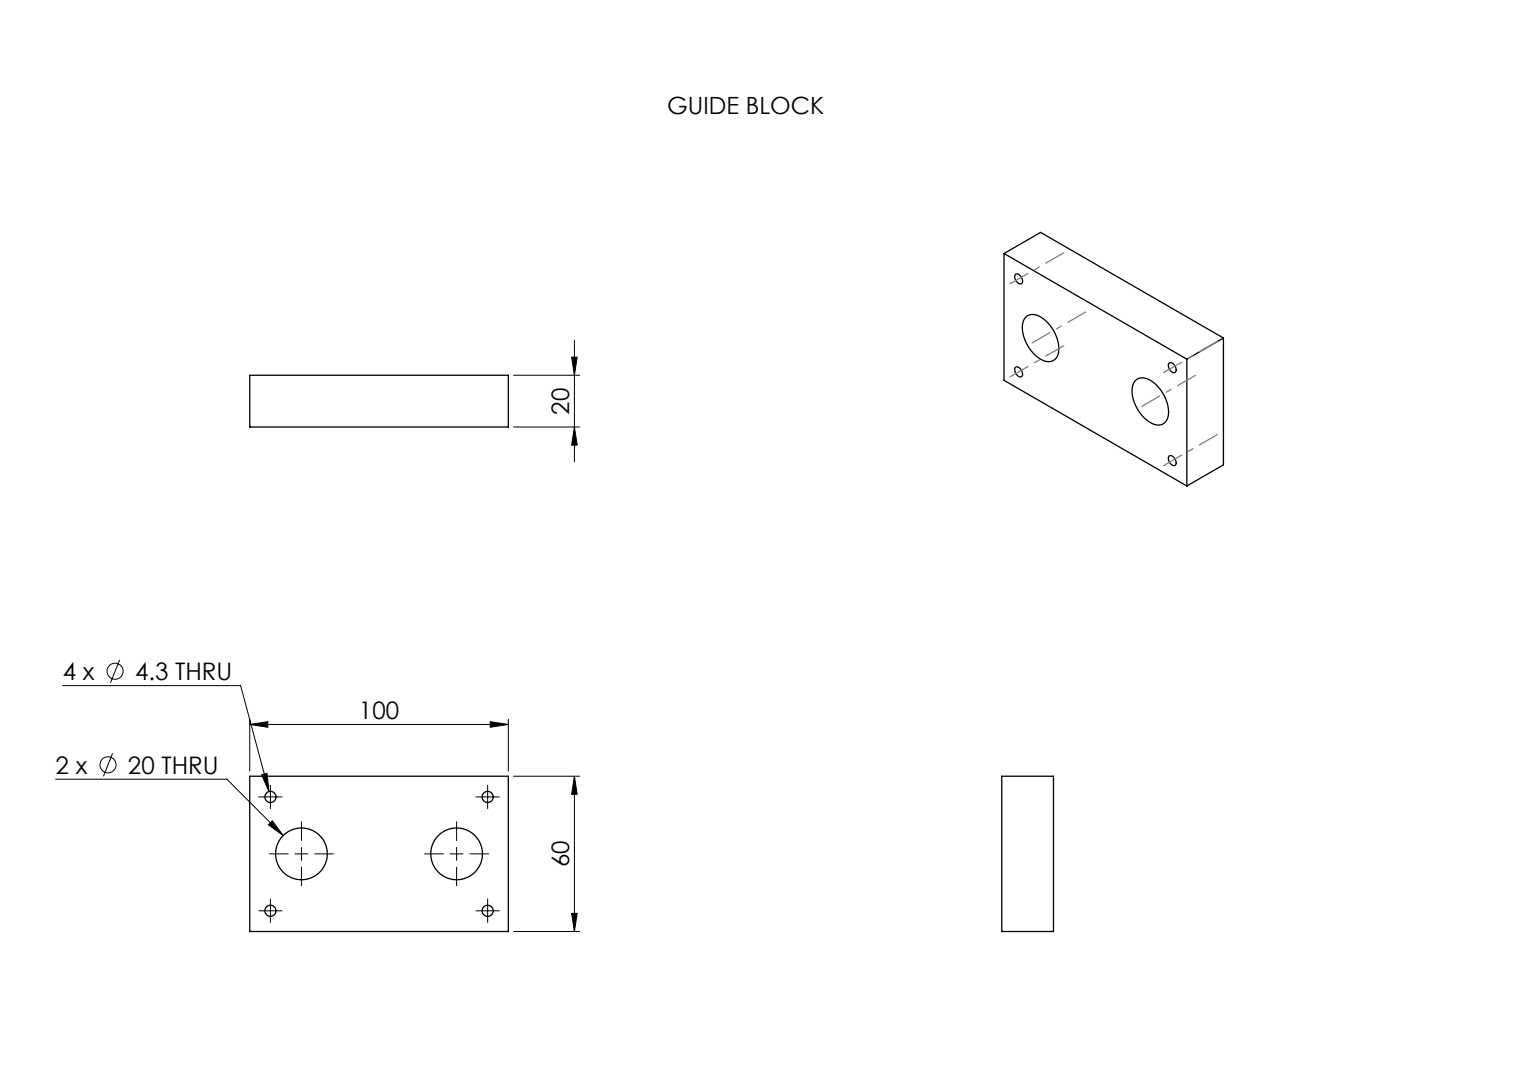
ISO-10303-21;
HEADER;
FILE_DESCRIPTION (('STEP AP214'),
    '1' );
FILE_NAME ('guide block.step',
    '2026-09-29T11:11:29',
    ( '' ),
    ( '' ),
    'SwSTEP 2.0',
    'SolidWorks 2026',
    '' );
FILE_SCHEMA (( 'AUTOMOTIVE_DESIGN' ));
ENDSEC;

DATA;
#8=ADVANCED_FACE ( 'NONE', ( #3264 ), #5944, .F. ) ;
#9=FACE_BOUND ( 'NONE', #6715, .T. ) ;
#15=ORIENTED_EDGE ( 'NONE', *, *, #7694, .T. ) ;
#24=ADVANCED_BREP_SHAPE_REPRESENTATION ( '', ( #85, #2554 ), #7190 ) ;
#41=EDGE_CURVE ( 'NONE', #505, #4648, #4851, .T. ) ;
#48=EDGE_LOOP ( 'NONE', ( #5523, #4308 ) ) ;
#49=CARTESIAN_POINT ( 'NONE',  ( -41.99999999999996447, -22.00000000000000000, 80.00000000000002842 ) ) ;
#67=CARTESIAN_POINT ( 'NONE',  ( 42.00000000000000711, -21.99999999999992184, 80.00000000000002842 ) ) ;
#74=AXIS2_PLACEMENT_3D ( 'NONE', #4907, #6141, #4116 ) ;
#80=DIRECTION ( 'NONE',  ( 1.000000000000000000, 0.000000000000000000, 0.000000000000000000 ) ) ;
#83=AXIS2_PLACEMENT_3D ( 'NONE', #2600, #8057, #1442 ) ;
#85=MANIFOLD_SOLID_BREP ( '\X2\00d8\X0\20.0 (20) Diameter Hole1', #4490 ) ;
#108=ORIENTED_EDGE ( 'NONE', *, *, #689, .F. ) ;
#120=VERTEX_POINT ( 'NONE', #6909 ) ;
#143=CIRCLE ( 'NONE', #4647, 9.999999999999998224 ) ;
#177=ADVANCED_FACE ( 'NONE', ( #4445 ), #1804, .F. ) ;
#184=LINE ( 'NONE', #7585, #2081 ) ;
#191=DIRECTION ( 'NONE',  ( -0.000000000000000000, 0.000000000000000000, 1.000000000000000000 ) ) ;
#212=SURFACE_SIDE_STYLE ('',( #6821 ) ) ;
#226=DIRECTION ( 'NONE',  ( -0.000000000000000000, -0.000000000000000000, -1.000000000000000000 ) ) ;
#231=CARTESIAN_POINT ( 'NONE',  ( -30.00000000000000000, 0.000000000000000000, 80.00000000000002842 ) ) ;
#234=EDGE_LOOP ( 'NONE', ( #2783, #7992, #7432, #4971 ) ) ;
#240=AXIS2_PLACEMENT_3D ( 'NONE', #1947, #6742, #7321 ) ;
#242=( GEOMETRIC_REPRESENTATION_CONTEXT ( 3 ) GLOBAL_UNCERTAINTY_ASSIGNED_CONTEXT ( ( #3453 ) ) GLOBAL_UNIT_ASSIGNED_CONTEXT ( ( #4314, #5632, #8331 ) ) REPRESENTATION_CONTEXT ( 'NONE', 'WORKASPACE' ) );
#250=EDGE_CURVE ( 'NONE', #6544, #5958, #4898, .T. ) ;
#273=DIRECTION ( 'NONE',  ( -0.000000000000000000, -0.000000000000000000, 1.000000000000000000 ) ) ;
#275=EDGE_CURVE ( 'NONE', #5958, #6544, #655, .T. ) ;
#293=EDGE_LOOP ( 'NONE', ( #5848, #7323 ) ) ;
#312=AXIS2_PLACEMENT_3D ( 'NONE', #7185, #3059, #1145 ) ;
#316=CARTESIAN_POINT ( 'NONE',  ( -39.84999999999998010, -22.00000000000000000, 80.00000000000002842 ) ) ;
#317=CARTESIAN_POINT ( 'NONE',  ( 39.85000000000002274, 21.99999999999992184, 60.00000000000002842 ) ) ;
#350=LINE ( 'NONE', #3185, #3142 ) ;
#368=AXIS2_PLACEMENT_3D ( 'NONE', #2667, #5963, #5335 ) ;
#380=LINE ( 'NONE', #8542, #1299 ) ;
#382=DIRECTION ( 'NONE',  ( -0.000000000000000000, 0.000000000000000000, 1.000000000000000000 ) ) ;
#406=DIRECTION ( 'NONE',  ( 1.000000000000000000, 0.000000000000000000, 0.000000000000000000 ) ) ;
#436=ORIENTED_EDGE ( 'NONE', *, *, #4043, .T. ) ;
#446=DIRECTION ( 'NONE',  ( 1.000000000000000000, 0.000000000000000000, 0.000000000000000000 ) ) ;
#459=DIRECTION ( 'NONE',  ( -0.000000000000000000, -0.000000000000000000, 1.000000000000000000 ) ) ;
#483=PLANE ( 'NONE',  #6432 ) ;
#490=( LENGTH_UNIT ( ) NAMED_UNIT ( * ) SI_UNIT ( .MILLI., .METRE. ) );
#504=EDGE_CURVE ( 'NONE', #3192, #4124, #958, .T. ) ;
#505=VERTEX_POINT ( 'NONE', #7187 ) ;
#517=AXIS2_PLACEMENT_3D ( 'NONE', #552, #1736, #7060 ) ;
#542=ORIENTED_EDGE ( 'NONE', *, *, #7814, .F. ) ;
#544=CARTESIAN_POINT ( 'NONE',  ( -39.99999999999999289, 1.224646799147353059E-15, 60.00000000000002842 ) ) ;
#545=CARTESIAN_POINT ( 'NONE',  ( -44.14999999999995595, 22.00000000000000000, 60.00000000000002842 ) ) ;
#549=CARTESIAN_POINT ( 'NONE',  ( -50.00000000000002842, -30.00000000000000000, 60.00000000000002842 ) ) ;
#552=CARTESIAN_POINT ( 'NONE',  ( 42.00000000000000711, 21.99999999999992184, 60.00000000000002842 ) ) ;
#560=AXIS2_PLACEMENT_3D ( 'NONE', #4014, #4102, #4307 ) ;
#576=CARTESIAN_POINT ( 'NONE',  ( 42.00000000000000711, -21.99999999999992184, 80.00000000000002842 ) ) ;
#608=UNCERTAINTY_MEASURE_WITH_UNIT (LENGTH_MEASURE( 1.000000000000000082E-05 ), #1837, 'distance_accuracy_value', 'NONE');
#623=DIRECTION ( 'NONE',  ( -1.000000000000000000, -0.000000000000000000, -0.000000000000000000 ) ) ;
#642=ORIENTED_EDGE ( 'NONE', *, *, #4452, .F. ) ;
#655=CIRCLE ( 'NONE', #1387, 2.149999999999985256 ) ;
#662=DIRECTION ( 'NONE',  ( 1.000000000000000000, 0.000000000000000000, 0.000000000000000000 ) ) ;
#667=FACE_BOUND ( 'NONE', #7929, .T. ) ;
#670=DIRECTION ( 'NONE',  ( -0.000000000000000000, -0.000000000000000000, 1.000000000000000000 ) ) ;
#680=ORIENTED_EDGE ( 'NONE', *, *, #275, .T. ) ;
#684=CARTESIAN_POINT ( 'NONE',  ( 29.99999999999997158, 1.102182119232617753E-14, 80.00000000000002842 ) ) ;
#689=EDGE_CURVE ( 'NONE', #4311, #8113, #1014, .T. ) ;
#703=LINE ( 'NONE', #3322, #4754 ) ;
#738=ORIENTED_EDGE ( 'NONE', *, *, #5306, .T. ) ;
#770=ORIENTED_EDGE ( 'NONE', *, *, #6382, .T. ) ;
#779=EDGE_LOOP ( 'NONE', ( #8638, #5179, #3636, #2635 ) ) ;
#831=DIRECTION ( 'NONE',  ( -0.000000000000000000, 0.000000000000000000, 1.000000000000000000 ) ) ;
#851=ORIENTED_EDGE ( 'NONE', *, *, #4407, .F. ) ;
#865=( GEOMETRIC_REPRESENTATION_CONTEXT ( 3 ) GLOBAL_UNCERTAINTY_ASSIGNED_CONTEXT ( ( #8028 ) ) GLOBAL_UNIT_ASSIGNED_CONTEXT ( ( #490, #6581, #1919 ) ) REPRESENTATION_CONTEXT ( 'NONE', 'WORKASPACE' ) );
#871=CARTESIAN_POINT ( 'NONE',  ( 50.00000000000002842, 30.00000000000000000, 80.00000000000002842 ) ) ;
#874=CARTESIAN_POINT ( 'NONE',  ( -41.99999999999996447, 22.00000000000000000, 60.00000000000002842 ) ) ;
#878=CIRCLE ( 'NONE', #6363, 2.149999999999985256 ) ;
#890=LINE ( 'NONE', #8264, #2347 ) ;
#894=CARTESIAN_POINT ( 'NONE',  ( 19.99999999999997513, 1.224646799147352901E-14, 60.00000000000002842 ) ) ;
#904=ADVANCED_FACE ( 'NONE', ( #6066 ), #8012, .F. ) ;
#923=VERTEX_POINT ( 'NONE', #545 ) ;
#936=FACE_OUTER_BOUND ( 'NONE', #5015, .T. ) ;
#938=DIRECTION ( 'NONE',  ( -0.000000000000000000, -0.000000000000000000, -1.000000000000000000 ) ) ;
#949=DIRECTION ( 'NONE',  ( -0.000000000000000000, -0.000000000000000000, 1.000000000000000000 ) ) ;
#958=CIRCLE ( 'NONE', #517, 2.149999999999985256 ) ;
#994=ORIENTED_EDGE ( 'NONE', *, *, #4575, .T. ) ;
#1001=DIRECTION ( 'NONE',  ( 1.000000000000000000, 0.000000000000000000, 0.000000000000000000 ) ) ;
#1014=CIRCLE ( 'NONE', #1437, 9.999999999999994671 ) ;
#1030=AXIS2_PLACEMENT_3D ( 'NONE', #3905, #1084, #4520 ) ;
#1060=VECTOR ( 'NONE', #1897, 1000.000000000000000 ) ;
#1084=DIRECTION ( 'NONE',  ( -0.000000000000000000, 0.000000000000000000, 1.000000000000000000 ) ) ;
#1087=VECTOR ( 'NONE', #7029, 1000.000000000000000 ) ;
#1104=DIRECTION ( 'NONE',  ( 1.000000000000000000, 0.000000000000000000, 0.000000000000000000 ) ) ;
#1108=LINE ( 'NONE', #2483, #4639 ) ;
#1109=LINE ( 'NONE', #3152, #4900 ) ;
#1130=CIRCLE ( 'NONE', #6474, 2.149999999999985256 ) ;
#1131=DIRECTION ( 'NONE',  ( -0.000000000000000000, 0.000000000000000000, 1.000000000000000000 ) ) ;
#1136=ORIENTED_EDGE ( 'NONE', *, *, #41, .T. ) ;
#1145=DIRECTION ( 'NONE',  ( 1.000000000000000000, 0.000000000000000000, 0.000000000000000000 ) ) ;
#1159=LINE ( 'NONE', #7780, #1087 ) ;
#1168=CARTESIAN_POINT ( 'NONE',  ( 44.14999999999999147, 21.99999999999992184, 60.00000000000002842 ) ) ;
#1200=PLANE ( 'NONE',  #368 ) ;
#1205=LINE ( 'NONE', #5255, #2854 ) ;
#1230=DIRECTION ( 'NONE',  ( 0.000000000000000000, -1.000000000000000000, 0.000000000000000000 ) ) ;
#1248=SHAPE_REPRESENTATION_RELATIONSHIP ( 'NONE' , 'NONE' ,  #4396, #24 ) ;
#1276=MECHANICAL_DESIGN_GEOMETRIC_PRESENTATION_REPRESENTATION('',(#2556),#865);
#1291=DIRECTION ( 'NONE',  ( 0.000000000000000000, -1.000000000000000000, 0.000000000000000000 ) ) ;
#1297=VERTEX_POINT ( 'NONE', #2924 ) ;
#1299=VECTOR ( 'NONE', #459, 1000.000000000000000 ) ;
#1350=ORIENTED_EDGE ( 'NONE', *, *, #250, .T. ) ;
#1371=ORIENTED_EDGE ( 'NONE', *, *, #3878, .F. ) ;
#1375=CYLINDRICAL_SURFACE ( 'NONE', #4181, 9.999999999999994671 ) ;
#1376=CARTESIAN_POINT ( 'NONE',  ( -40.00000000000000000, 1.224646799147353454E-15, 80.00000000000002842 ) ) ;
#1381=FILL_AREA_STYLE_COLOUR ( '', #8474 ) ;
#1383=CARTESIAN_POINT ( 'NONE',  ( -41.99999999999996447, 22.00000000000000000, 80.00000000000002842 ) ) ;
#1387=AXIS2_PLACEMENT_3D ( 'NONE', #3825, #5720, #7090 ) ;
#1416=FACE_BOUND ( 'NONE', #1448, .T. ) ;
#1418=EDGE_CURVE ( 'NONE', #7457, #2517, #6025, .T. ) ;
#1421=EDGE_CURVE ( 'NONE', #2540, #2072, #5423, .T. ) ;
#1428=PLANE ( 'NONE',  #6426 ) ;
#1434=VERTEX_POINT ( 'NONE', #549 ) ;
#1437=AXIS2_PLACEMENT_3D ( 'NONE', #3049, #3701, #6381 ) ;
#1442=DIRECTION ( 'NONE',  ( 0.000000000000000000, -0.000000000000000000, 1.000000000000000000 ) ) ;
#1444=ADVANCED_FACE ( 'NONE', ( #7394 ), #5354, .F. ) ;
#1448=EDGE_LOOP ( 'NONE', ( #7819, #5270 ) ) ;
#1506=AXIS2_PLACEMENT_3D ( 'NONE', #1715, #5676, #1001 ) ;
#1550=DIRECTION ( 'NONE',  ( -0.000000000000000000, -0.000000000000000000, 1.000000000000000000 ) ) ;
#1576=PRODUCT_DEFINITION ( 'UNKNOWN', '', #3409, #8552 ) ;
#1595=CYLINDRICAL_SURFACE ( 'NONE', #74, 9.999999999999994671 ) ;
#1627=ORIENTED_EDGE ( 'NONE', *, *, #6127, .F. ) ;
#1635=VECTOR ( 'NONE', #5981, 1000.000000000000000 ) ;
#1685=CARTESIAN_POINT ( 'NONE',  ( -50.00000000000002842, -30.00000000000000000, 60.00000000000002842 ) ) ;
#1707=DIRECTION ( 'NONE',  ( 0.000000000000000000, 0.000000000000000000, 1.000000000000000000 ) ) ;
#1712=AXIS2_PLACEMENT_3D ( 'NONE', #6266, #5601, #7672 ) ;
#1715=CARTESIAN_POINT ( 'NONE',  ( -41.99999999999996447, 22.00000000000000000, 80.00000000000002842 ) ) ;
#1736=DIRECTION ( 'NONE',  ( -0.000000000000000000, 0.000000000000000000, 1.000000000000000000 ) ) ;
#1737=DIRECTION ( 'NONE',  ( 1.000000000000000000, 0.000000000000000000, 0.000000000000000000 ) ) ;
#1745=ORIENTED_EDGE ( 'NONE', *, *, #41, .F. ) ;
#1761=ORIENTED_EDGE ( 'NONE', *, *, #5886, .T. ) ;
#1778=LINE ( 'NONE', #4007, #5943 ) ;
#1780=CARTESIAN_POINT ( 'NONE',  ( 42.00000000000000711, -21.99999999999992184, 80.00000000000002842 ) ) ;
#1802=MECHANICAL_DESIGN_GEOMETRIC_PRESENTATION_REPRESENTATION('',(#7848),#242);
#1804=CYLINDRICAL_SURFACE ( 'NONE', #1506, 2.149999999999985256 ) ;
#1811=ORIENTED_EDGE ( 'NONE', *, *, #5412, .T. ) ;
#1818=ADVANCED_FACE ( 'NONE', ( #6047 ), #1375, .F. ) ;
#1836=ADVANCED_FACE ( 'NONE', ( #7327, #2622, #667, #5251, #9, #3418, #8694 ), #1200, .T. ) ;
#1837=( LENGTH_UNIT ( ) NAMED_UNIT ( * ) SI_UNIT ( .MILLI., .METRE. ) );
#1854=EDGE_CURVE ( 'NONE', #7457, #1434, #7240, .T. ) ;
#1886=ORIENTED_EDGE ( 'NONE', *, *, #4542, .F. ) ;
#1887=VERTEX_POINT ( 'NONE', #1954 ) ;
#1894=ORIENTED_EDGE ( 'NONE', *, *, #4940, .T. ) ;
#1897=DIRECTION ( 'NONE',  ( 1.000000000000000000, 0.000000000000000000, 0.000000000000000000 ) ) ;
#1911=AXIS2_PLACEMENT_3D ( 'NONE', #3063, #5945, #1737 ) ;
#1919=( NAMED_UNIT ( * ) SI_UNIT ( $, .STERADIAN. ) SOLID_ANGLE_UNIT ( ) );
#1929=DIRECTION ( 'NONE',  ( -0.000000000000000000, -0.000000000000000000, 1.000000000000000000 ) ) ;
#1947=CARTESIAN_POINT ( 'NONE',  ( 29.99999999999997158, 1.102182119232617753E-14, 60.00000000000002842 ) ) ;
#1950=ORIENTED_EDGE ( 'NONE', *, *, #3451, .T. ) ;
#1954=CARTESIAN_POINT ( 'NONE',  ( 44.14999999999999147, 21.99999999999992184, 80.00000000000002842 ) ) ;
#1988=EDGE_CURVE ( 'NONE', #4697, #4311, #890, .T. ) ;
#2007=ORIENTED_EDGE ( 'NONE', *, *, #3451, .F. ) ;
#2008=DIRECTION ( 'NONE',  ( -0.000000000000000000, -0.000000000000000000, 1.000000000000000000 ) ) ;
#2014=EDGE_LOOP ( 'NONE', ( #6914, #542 ) ) ;
#2020=DIRECTION ( 'NONE',  ( 1.000000000000000000, 0.000000000000000000, 0.000000000000000000 ) ) ;
#2021=DIRECTION ( 'NONE',  ( -0.000000000000000000, 0.000000000000000000, 1.000000000000000000 ) ) ;
#2026=ADVANCED_FACE ( 'NONE', ( #6094 ), #1595, .F. ) ;
#2037=CARTESIAN_POINT ( 'NONE',  ( 39.85000000000002274, 21.99999999999992184, 80.00000000000002842 ) ) ;
#2051=SURFACE_STYLE_FILL_AREA ( #5299 ) ;
#2071=ORIENTED_EDGE ( 'NONE', *, *, #4679, .T. ) ;
#2072=VERTEX_POINT ( 'NONE', #5467 ) ;
#2081=VECTOR ( 'NONE', #226, 1000.000000000000000 ) ;
#2088=ORIENTED_EDGE ( 'NONE', *, *, #4214, .T. ) ;
#2108=ORIENTED_EDGE ( 'NONE', *, *, #5306, .F. ) ;
#2120=FILL_AREA_STYLE_COLOUR ( '', #3766 ) ;
#2129=CIRCLE ( 'NONE', #2684, 2.149999999999985256 ) ;
#2187=ORIENTED_EDGE ( 'NONE', *, *, #4214, .F. ) ;
#2189=ORIENTED_EDGE ( 'NONE', *, *, #504, .F. ) ;
#2229=CARTESIAN_POINT ( 'NONE',  ( 42.00000000000000711, 21.99999999999992184, 80.00000000000002842 ) ) ;
#2252=DIRECTION ( 'NONE',  ( -0.000000000000000000, -0.000000000000000000, -1.000000000000000000 ) ) ;
#2277=LINE ( 'NONE', #3144, #7975 ) ;
#2286=EDGE_CURVE ( 'NONE', #5578, #7382, #6687, .T. ) ;
#2302=VERTEX_POINT ( 'NONE', #316 ) ;
#2304=CIRCLE ( 'NONE', #5111, 9.999999999999994671 ) ;
#2313=EDGE_CURVE ( 'NONE', #1434, #120, #8639, .T. ) ;
#2323=VERTEX_POINT ( 'NONE', #2400 ) ;
#2347=VECTOR ( 'NONE', #1550, 1000.000000000000000 ) ;
#2386=DIRECTION ( 'NONE',  ( 1.000000000000000000, 0.000000000000000000, 0.000000000000000000 ) ) ;
#2400=CARTESIAN_POINT ( 'NONE',  ( 39.85000000000002274, -21.99999999999992184, 80.00000000000002842 ) ) ;
#2404=CARTESIAN_POINT ( 'NONE',  ( -39.84999999999998010, 22.00000000000000000, 60.00000000000002842 ) ) ;
#2413=DIRECTION ( 'NONE',  ( 1.000000000000000000, 0.000000000000000000, 0.000000000000000000 ) ) ;
#2437=CARTESIAN_POINT ( 'NONE',  ( -30.00000000000000000, 0.000000000000000000, 60.00000000000002842 ) ) ;
#2442=CARTESIAN_POINT ( 'NONE',  ( 44.14999999999999147, -21.99999999999992184, 80.00000000000002842 ) ) ;
#2446=CIRCLE ( 'NONE', #1030, 9.999999999999994671 ) ;
#2447=ORIENTED_EDGE ( 'NONE', *, *, #4575, .F. ) ;
#2476=VECTOR ( 'NONE', #6589, 1000.000000000000000 ) ;
#2480=CYLINDRICAL_SURFACE ( 'NONE', #312, 2.149999999999985256 ) ;
#2483=CARTESIAN_POINT ( 'NONE',  ( 44.14999999999999147, 21.99999999999992184, 80.00000000000002842 ) ) ;
#2490=EDGE_CURVE ( 'NONE', #2072, #2323, #4529, .T. ) ;
#2496=EDGE_CURVE ( 'NONE', #923, #7483, #380, .T. ) ;
#2506=VERTEX_POINT ( 'NONE', #544 ) ;
#2517=VERTEX_POINT ( 'NONE', #8582 ) ;
#2540=VERTEX_POINT ( 'NONE', #4403 ) ;
#2545=EDGE_LOOP ( 'NONE', ( #6333, #1745, #2108, #1761 ) ) ;
#2554=AXIS2_PLACEMENT_3D ( 'NONE', #7787, #1707, #3692 ) ;
#2556=STYLED_ITEM ( 'NONE', ( #4564 ), #24 ) ;
#2593=ORIENTED_EDGE ( 'NONE', *, *, #8199, .F. ) ;
#2597=DIRECTION ( 'NONE',  ( -0.000000000000000000, -0.000000000000000000, 1.000000000000000000 ) ) ;
#2600=CARTESIAN_POINT ( 'NONE',  ( -50.00000000000002842, -30.00000000000000000, 80.00000000000002842 ) ) ;
#2604=ORIENTED_EDGE ( 'NONE', *, *, #275, .F. ) ;
#2618=FACE_BOUND ( 'NONE', #8172, .T. ) ;
#2622=FACE_BOUND ( 'NONE', #7527, .T. ) ;
#2628=( NAMED_UNIT ( * ) SI_UNIT ( $, .STERADIAN. ) SOLID_ANGLE_UNIT ( ) );
#2635=ORIENTED_EDGE ( 'NONE', *, *, #7694, .F. ) ;
#2636=ORIENTED_EDGE ( 'NONE', *, *, #6281, .F. ) ;
#2667=CARTESIAN_POINT ( 'NONE',  ( 0.000000000000000000, 0.000000000000000000, 80.00000000000002842 ) ) ;
#2670=CARTESIAN_POINT ( 'NONE',  ( -39.84999999999998010, -22.00000000000000000, 80.00000000000002842 ) ) ;
#2680=EDGE_LOOP ( 'NONE', ( #738, #1950, #2716, #5385 ) ) ;
#2684=AXIS2_PLACEMENT_3D ( 'NONE', #7741, #7080, #446 ) ;
#2712=DIRECTION ( 'NONE',  ( -0.000000000000000000, -0.000000000000000000, 1.000000000000000000 ) ) ;
#2716=ORIENTED_EDGE ( 'NONE', *, *, #4452, .T. ) ;
#2745=ADVANCED_FACE ( 'NONE', ( #6021 ), #7434, .F. ) ;
#2753=DIRECTION ( 'NONE',  ( -0.000000000000000000, -0.000000000000000000, 1.000000000000000000 ) ) ;
#2783=ORIENTED_EDGE ( 'NONE', *, *, #4976, .F. ) ;
#2794=SHAPE_DEFINITION_REPRESENTATION ( #8394, #4396 ) ;
#2819=ORIENTED_EDGE ( 'NONE', *, *, #4417, .F. ) ;
#2824=AXIS2_PLACEMENT_3D ( 'NONE', #8000, #2712, #8617 ) ;
#2847=DIRECTION ( 'NONE',  ( -0.000000000000000000, -0.000000000000000000, 1.000000000000000000 ) ) ;
#2854=VECTOR ( 'NONE', #7379, 1000.000000000000000 ) ;
#2868=CIRCLE ( 'NONE', #4543, 2.149999999999985256 ) ;
#2896=ORIENTED_EDGE ( 'NONE', *, *, #5886, .F. ) ;
#2913=ORIENTED_EDGE ( 'NONE', *, *, #8104, .F. ) ;
#2924=CARTESIAN_POINT ( 'NONE',  ( -50.00000000000002842, 30.00000000000000000, 60.00000000000002842 ) ) ;
#2930=EDGE_CURVE ( 'NONE', #5183, #1887, #2868, .T. ) ;
#2934=CARTESIAN_POINT ( 'NONE',  ( -50.00000000000002842, 30.00000000000000000, 80.00000000000002842 ) ) ;
#2952=AXIS2_PLACEMENT_3D ( 'NONE', #3355, #5272, #6641 ) ;
#2957=PRESENTATION_STYLE_ASSIGNMENT (( #4802 ) ) ;
#3017=CARTESIAN_POINT ( 'NONE',  ( -39.84999999999998010, 22.00000000000000000, 80.00000000000002842 ) ) ;
#3049=CARTESIAN_POINT ( 'NONE',  ( 29.99999999999997158, 1.102182119232617753E-14, 80.00000000000002842 ) ) ;
#3054=ORIENTED_EDGE ( 'NONE', *, *, #8104, .T. ) ;
#3059=DIRECTION ( 'NONE',  ( -0.000000000000000000, -0.000000000000000000, 1.000000000000000000 ) ) ;
#3063=CARTESIAN_POINT ( 'NONE',  ( -30.00000000000000000, 0.000000000000000000, 80.00000000000002842 ) ) ;
#3064=DIRECTION ( 'NONE',  ( -0.000000000000000000, -0.000000000000000000, 1.000000000000000000 ) ) ;
#3116=DIRECTION ( 'NONE',  ( -1.000000000000000000, 0.000000000000000000, 0.000000000000000000 ) ) ;
#3138=EDGE_CURVE ( 'NONE', #2506, #6156, #2446, .T. ) ;
#3142=VECTOR ( 'NONE', #5736, 1000.000000000000000 ) ;
#3144=CARTESIAN_POINT ( 'NONE',  ( -50.00000000000002842, 30.00000000000000000, 80.00000000000002842 ) ) ;
#3147=AXIS2_PLACEMENT_3D ( 'NONE', #5871, #5914, #3976 ) ;
#3152=CARTESIAN_POINT ( 'NONE',  ( 50.00000000000002842, 30.00000000000000000, 60.00000000000002842 ) ) ;
#3185=CARTESIAN_POINT ( 'NONE',  ( 39.85000000000002274, 21.99999999999992184, 80.00000000000002842 ) ) ;
#3192=VERTEX_POINT ( 'NONE', #1168 ) ;
#3203=LINE ( 'NONE', #7912, #4711 ) ;
#3246=( NAMED_UNIT ( * ) PLANE_ANGLE_UNIT ( ) SI_UNIT ( $, .RADIAN. ) );
#3264=FACE_OUTER_BOUND ( 'NONE', #7296, .T. ) ;
#3291=DIRECTION ( 'NONE',  ( 1.000000000000000000, 0.000000000000000000, 0.000000000000000000 ) ) ;
#3295=SURFACE_SIDE_STYLE ('',( #2051 ) ) ;
#3308=AXIS2_PLACEMENT_3D ( 'NONE', #6496, #5711, #406 ) ;
#3322=CARTESIAN_POINT ( 'NONE',  ( 50.00000000000002842, 30.00000000000000000, 80.00000000000002842 ) ) ;
#3326=CYLINDRICAL_SURFACE ( 'NONE', #8419, 2.149999999999985256 ) ;
#3349=ADVANCED_FACE ( 'NONE', ( #5970 ), #1428, .F. ) ;
#3355=CARTESIAN_POINT ( 'NONE',  ( -30.00000000000000000, 0.000000000000000000, 80.00000000000002842 ) ) ;
#3380=CARTESIAN_POINT ( 'NONE',  ( -50.00000000000002842, 30.00000000000000000, 80.00000000000002842 ) ) ;
#3384=EDGE_CURVE ( 'NONE', #5890, #7483, #4317, .T. ) ;
#3385=ORIENTED_EDGE ( 'NONE', *, *, #5412, .F. ) ;
#3409=PRODUCT_DEFINITION_FORMATION_WITH_SPECIFIED_SOURCE ( 'ANY', '', #7676, .NOT_KNOWN. ) ;
#3418=FACE_BOUND ( 'NONE', #293, .T. ) ;
#3451=EDGE_CURVE ( 'NONE', #505, #4683, #2277, .T. ) ;
#3453=UNCERTAINTY_MEASURE_WITH_UNIT (LENGTH_MEASURE( 1.000000000000000082E-05 ), #4314, 'distance_accuracy_value', 'NONE');
#3494=CIRCLE ( 'NONE', #240, 9.999999999999994671 ) ;
#3509=CARTESIAN_POINT ( 'NONE',  ( 50.00000000000002842, 30.00000000000000000, 60.00000000000002842 ) ) ;
#3527=ORIENTED_EDGE ( 'NONE', *, *, #4675, .T. ) ;
#3536=AXIS2_PLACEMENT_3D ( 'NONE', #4910, #191, #6314 ) ;
#3546=CYLINDRICAL_SURFACE ( 'NONE', #4500, 2.149999999999985256 ) ;
#3548=DIRECTION ( 'NONE',  ( -0.000000000000000000, -0.000000000000000000, 1.000000000000000000 ) ) ;
#3561=CIRCLE ( 'NONE', #8484, 2.149999999999985256 ) ;
#3594=LINE ( 'NONE', #6098, #3719 ) ;
#3596=DIRECTION ( 'NONE',  ( -0.000000000000000000, -0.000000000000000000, 1.000000000000000000 ) ) ;
#3630=CARTESIAN_POINT ( 'NONE',  ( -39.99999999999999289, 1.224646799147352862E-15, 80.00000000000002842 ) ) ;
#3636=ORIENTED_EDGE ( 'NONE', *, *, #689, .T. ) ;
#3651=ADVANCED_FACE ( 'NONE', ( #7021 ), #4957, .F. ) ;
#3692=DIRECTION ( 'NONE',  ( 1.000000000000000000, 0.000000000000000000, 0.000000000000000000 ) ) ;
#3701=DIRECTION ( 'NONE',  ( -0.000000000000000000, -0.000000000000000000, 1.000000000000000000 ) ) ;
#3717=CYLINDRICAL_SURFACE ( 'NONE', #8169, 2.149999999999985256 ) ;
#3719=VECTOR ( 'NONE', #2847, 1000.000000000000000 ) ;
#3766=COLOUR_RGB ( '', 0.09019608, 0.27058824, 0.51372549) ;
#3798=VECTOR ( 'NONE', #273, 1000.000000000000000 ) ;
#3823=ORIENTED_EDGE ( 'NONE', *, *, #7586, .T. ) ;
#3825=CARTESIAN_POINT ( 'NONE',  ( -41.99999999999996447, -22.00000000000000000, 60.00000000000002842 ) ) ;
#3835=CARTESIAN_POINT ( 'NONE',  ( -44.14999999999995595, -22.00000000000000000, 80.00000000000002842 ) ) ;
#3836=ADVANCED_FACE ( 'NONE', ( #6798 ), #3546, .F. ) ;
#3838=CARTESIAN_POINT ( 'NONE',  ( -20.00000000000000355, 0.000000000000000000, 60.00000000000002842 ) ) ;
#3855=FACE_OUTER_BOUND ( 'NONE', #2545, .T. ) ;
#3875=DIRECTION ( 'NONE',  ( 1.000000000000000000, 0.000000000000000000, 0.000000000000000000 ) ) ;
#3878=EDGE_CURVE ( 'NONE', #6156, #7382, #7545, .T. ) ;
#3895=DIRECTION ( 'NONE',  ( -0.000000000000000000, -0.000000000000000000, -1.000000000000000000 ) ) ;
#3904=EDGE_LOOP ( 'NONE', ( #8667, #2896, #5028, #8192 ) ) ;
#3905=CARTESIAN_POINT ( 'NONE',  ( -30.00000000000000000, 0.000000000000000000, 60.00000000000002842 ) ) ;
#3932=CARTESIAN_POINT ( 'NONE',  ( -41.99999999999996447, -22.00000000000000000, 80.00000000000002842 ) ) ;
#3938=CIRCLE ( 'NONE', #2824, 2.149999999999985256 ) ;
#3943=ADVANCED_FACE ( 'NONE', ( #936 ), #3717, .F. ) ;
#3976=DIRECTION ( 'NONE',  ( -0.000000000000000000, 0.000000000000000000, -1.000000000000000000 ) ) ;
#3979=FACE_BOUND ( 'NONE', #5491, .T. ) ;
#3992=DIRECTION ( 'NONE',  ( 0.000000000000000000, -0.000000000000000000, -1.000000000000000000 ) ) ;
#4007=CARTESIAN_POINT ( 'NONE',  ( -39.84999999999998010, 22.00000000000000000, 80.00000000000002842 ) ) ;
#4014=CARTESIAN_POINT ( 'NONE',  ( 42.00000000000000711, 21.99999999999992184, 60.00000000000002842 ) ) ;
#4041=VERTEX_POINT ( 'NONE', #2442 ) ;
#4043=EDGE_CURVE ( 'NONE', #3192, #1887, #1108, .T. ) ;
#4102=DIRECTION ( 'NONE',  ( -0.000000000000000000, 0.000000000000000000, 1.000000000000000000 ) ) ;
#4106=EDGE_CURVE ( 'NONE', #2506, #5578, #6312, .T. ) ;
#4112=FACE_BOUND ( 'NONE', #7350, .T. ) ;
#4116=DIRECTION ( 'NONE',  ( 1.000000000000000000, 0.000000000000000000, 0.000000000000000000 ) ) ;
#4119=LINE ( 'NONE', #4161, #8176 ) ;
#4121=AXIS2_PLACEMENT_3D ( 'NONE', #8056, #5398, #2020 ) ;
#4124=VERTEX_POINT ( 'NONE', #317 ) ;
#4161=CARTESIAN_POINT ( 'NONE',  ( -50.00000000000002842, 30.00000000000000000, 80.00000000000002842 ) ) ;
#4181=AXIS2_PLACEMENT_3D ( 'NONE', #6706, #7997, #6663 ) ;
#4214=EDGE_CURVE ( 'NONE', #7483, #5890, #2129, .T. ) ;
#4239=CARTESIAN_POINT ( 'NONE',  ( 39.99999999999996447, 1.102182119232617753E-14, 80.00000000000002842 ) ) ;
#4253=ORIENTED_EDGE ( 'NONE', *, *, #2930, .T. ) ;
#4259=CARTESIAN_POINT ( 'NONE',  ( 42.00000000000000711, 21.99999999999992184, 80.00000000000002842 ) ) ;
#4265=ORIENTED_EDGE ( 'NONE', *, *, #2496, .F. ) ;
#4307=DIRECTION ( 'NONE',  ( 1.000000000000000000, 0.000000000000000000, 0.000000000000000000 ) ) ;
#4308=ORIENTED_EDGE ( 'NONE', *, *, #2286, .F. ) ;
#4311=VERTEX_POINT ( 'NONE', #5135 ) ;
#4314=( LENGTH_UNIT ( ) NAMED_UNIT ( * ) SI_UNIT ( .MILLI., .METRE. ) );
#4317=CIRCLE ( 'NONE', #5723, 2.149999999999985256 ) ;
#4318=DIRECTION ( 'NONE',  ( -0.000000000000000000, -0.000000000000000000, 1.000000000000000000 ) ) ;
#4321=ORIENTED_EDGE ( 'NONE', *, *, #504, .T. ) ;
#4332=VECTOR ( 'NONE', #7856, 1000.000000000000000 ) ;
#4385=EDGE_LOOP ( 'NONE', ( #6262, #5530, #4712, #6135 ) ) ;
#4396=SHAPE_REPRESENTATION ( 'guide block', ( #2554 ), #7190 ) ;
#4403=CARTESIAN_POINT ( 'NONE',  ( 44.14999999999999147, -21.99999999999992184, 60.00000000000002842 ) ) ;
#4407=EDGE_CURVE ( 'NONE', #6544, #2302, #6619, .T. ) ;
#4417=EDGE_CURVE ( 'NONE', #4041, #2323, #3938, .T. ) ;
#4445=FACE_OUTER_BOUND ( 'NONE', #4937, .T. ) ;
#4452=EDGE_CURVE ( 'NONE', #4683, #7457, #1205, .T. ) ;
#4472=DIRECTION ( 'NONE',  ( 0.000000000000000000, 0.000000000000000000, 1.000000000000000000 ) ) ;
#4478=EDGE_LOOP ( 'NONE', ( #5218, #4702, #5155, #1371 ) ) ;
#4490=CLOSED_SHELL ( 'NONE', ( #2026, #1818, #177, #6872, #3943, #3836, #5424, #3349, #7858, #1444, #1836, #5731, #3651, #2745, #5818, #6131, #904, #8 ) ) ;
#4500=AXIS2_PLACEMENT_3D ( 'NONE', #2229, #6227, #6143 ) ;
#4519=ORIENTED_EDGE ( 'NONE', *, *, #6729, .F. ) ;
#4520=DIRECTION ( 'NONE',  ( 1.000000000000000000, 0.000000000000000000, 0.000000000000000000 ) ) ;
#4529=LINE ( 'NONE', #5810, #2476 ) ;
#4542=EDGE_CURVE ( 'NONE', #2323, #4041, #1130, .T. ) ;
#4543=AXIS2_PLACEMENT_3D ( 'NONE', #4259, #949, #5008 ) ;
#4564=PRESENTATION_STYLE_ASSIGNMENT (( #7956 ) ) ;
#4575=EDGE_CURVE ( 'NONE', #4984, #923, #6899, .T. ) ;
#4599=CARTESIAN_POINT ( 'NONE',  ( -50.00000000000002842, -30.00000000000000000, 80.00000000000002842 ) ) ;
#4604=DIRECTION ( 'NONE',  ( -0.000000000000000000, -0.000000000000000000, 1.000000000000000000 ) ) ;
#4612=ORIENTED_EDGE ( 'NONE', *, *, #1988, .F. ) ;
#4616=DIRECTION ( 'NONE',  ( 1.000000000000000000, 0.000000000000000000, 0.000000000000000000 ) ) ;
#4632=DIRECTION ( 'NONE',  ( -0.000000000000000000, 1.000000000000000000, -0.000000000000000000 ) ) ;
#4633=FACE_OUTER_BOUND ( 'NONE', #7219, .T. ) ;
#4639=VECTOR ( 'NONE', #3064, 1000.000000000000000 ) ;
#4647=AXIS2_PLACEMENT_3D ( 'NONE', #231, #3548, #6800 ) ;
#4648=VERTEX_POINT ( 'NONE', #3509 ) ;
#4675=EDGE_CURVE ( 'NONE', #4683, #1297, #4119, .T. ) ;
#4679=EDGE_CURVE ( 'NONE', #7382, #5578, #143, .T. ) ;
#4681=DIRECTION ( 'NONE',  ( -0.000000000000000000, -0.000000000000000000, 1.000000000000000000 ) ) ;
#4683=VERTEX_POINT ( 'NONE', #2934 ) ;
#4697=VERTEX_POINT ( 'NONE', #894 ) ;
#4702=ORIENTED_EDGE ( 'NONE', *, *, #4106, .T. ) ;
#4711=VECTOR ( 'NONE', #623, 1000.000000000000000 ) ;
#4712=ORIENTED_EDGE ( 'NONE', *, *, #5404, .T. ) ;
#4727=PRODUCT_CONTEXT ( 'NONE', #7853, 'mechanical' ) ;
#4751=CARTESIAN_POINT ( 'NONE',  ( -50.00000000000002842, -30.00000000000000000, 80.00000000000002842 ) ) ;
#4754=VECTOR ( 'NONE', #4632, 1000.000000000000000 ) ;
#4758=ORIENTED_EDGE ( 'NONE', *, *, #5404, .F. ) ;
#4802=SURFACE_STYLE_USAGE ( .BOTH. , #212 ) ;
#4851=LINE ( 'NONE', #871, #7864 ) ;
#4854=DIRECTION ( 'NONE',  ( 1.000000000000000000, 0.000000000000000000, 0.000000000000000000 ) ) ;
#4898=CIRCLE ( 'NONE', #8684, 2.149999999999985256 ) ;
#4900=VECTOR ( 'NONE', #5081, 1000.000000000000000 ) ;
#4907=CARTESIAN_POINT ( 'NONE',  ( -30.00000000000000000, 0.000000000000000000, 80.00000000000002842 ) ) ;
#4910=CARTESIAN_POINT ( 'NONE',  ( -41.99999999999996447, 22.00000000000000000, 60.00000000000002842 ) ) ;
#4919=ORIENTED_EDGE ( 'NONE', *, *, #4043, .F. ) ;
#4937=EDGE_LOOP ( 'NONE', ( #2636, #7151, #2088, #1627 ) ) ;
#4940=EDGE_CURVE ( 'NONE', #5958, #8507, #7730, .T. ) ;
#4941=CIRCLE ( 'NONE', #560, 2.149999999999985256 ) ;
#4957=CYLINDRICAL_SURFACE ( 'NONE', #6556, 2.149999999999985256 ) ;
#4971=ORIENTED_EDGE ( 'NONE', *, *, #7586, .F. ) ;
#4976=EDGE_CURVE ( 'NONE', #120, #4648, #1109, .T. ) ;
#4977=ORIENTED_EDGE ( 'NONE', *, *, #8448, .T. ) ;
#4984=VERTEX_POINT ( 'NONE', #2404 ) ;
#5000=DIRECTION ( 'NONE',  ( -1.000000000000000000, -0.000000000000000000, -0.000000000000000000 ) ) ;
#5008=DIRECTION ( 'NONE',  ( 1.000000000000000000, 0.000000000000000000, 0.000000000000000000 ) ) ;
#5015=EDGE_LOOP ( 'NONE', ( #2593, #8416, #5193, #4758 ) ) ;
#5025=ORIENTED_EDGE ( 'NONE', *, *, #8591, .F. ) ;
#5028=ORIENTED_EDGE ( 'NONE', *, *, #1418, .F. ) ;
#5049=CARTESIAN_POINT ( 'NONE',  ( 29.99999999999997158, 1.102182119232617753E-14, 80.00000000000002842 ) ) ;
#5064=DIRECTION ( 'NONE',  ( 1.000000000000000000, 0.000000000000000000, 0.000000000000000000 ) ) ;
#5081=DIRECTION ( 'NONE',  ( -0.000000000000000000, 1.000000000000000000, -0.000000000000000000 ) ) ;
#5111=AXIS2_PLACEMENT_3D ( 'NONE', #6383, #382, #5064 ) ;
#5135=CARTESIAN_POINT ( 'NONE',  ( 19.99999999999997513, 1.224646799147352901E-14, 80.00000000000002842 ) ) ;
#5155=ORIENTED_EDGE ( 'NONE', *, *, #2286, .T. ) ;
#5177=CARTESIAN_POINT ( 'NONE',  ( -44.14999999999995595, 22.00000000000000000, 80.00000000000002842 ) ) ;
#5179=ORIENTED_EDGE ( 'NONE', *, *, #1988, .T. ) ;
#5183=VERTEX_POINT ( 'NONE', #2037 ) ;
#5193=ORIENTED_EDGE ( 'NONE', *, *, #4542, .T. ) ;
#5218=ORIENTED_EDGE ( 'NONE', *, *, #3138, .F. ) ;
#5227=FACE_OUTER_BOUND ( 'NONE', #7877, .T. ) ;
#5251=FACE_BOUND ( 'NONE', #2014, .T. ) ;
#5255=CARTESIAN_POINT ( 'NONE',  ( -50.00000000000002842, 30.00000000000000000, 80.00000000000002842 ) ) ;
#5270=ORIENTED_EDGE ( 'NONE', *, *, #8199, .T. ) ;
#5272=DIRECTION ( 'NONE',  ( -0.000000000000000000, -0.000000000000000000, 1.000000000000000000 ) ) ;
#5286=CARTESIAN_POINT ( 'NONE',  ( 0.000000000000000000, 0.000000000000000000, 60.00000000000002842 ) ) ;
#5294=EDGE_CURVE ( 'NONE', #4697, #7212, #3494, .T. ) ;
#5299=FILL_AREA_STYLE ('',( #1381 ) ) ;
#5306=EDGE_CURVE ( 'NONE', #2517, #505, #703, .T. ) ;
#5335=DIRECTION ( 'NONE',  ( 1.000000000000000000, 0.000000000000000000, 0.000000000000000000 ) ) ;
#5354=PLANE ( 'NONE',  #83 ) ;
#5356=ORIENTED_EDGE ( 'NONE', *, *, #6223, .F. ) ;
#5375=AXIS2_PLACEMENT_3D ( 'NONE', #3932, #4681, #7233 ) ;
#5385=ORIENTED_EDGE ( 'NONE', *, *, #1418, .T. ) ;
#5386=DIRECTION ( 'NONE',  ( 1.000000000000000000, 0.000000000000000000, 0.000000000000000000 ) ) ;
#5398=DIRECTION ( 'NONE',  ( -0.000000000000000000, -0.000000000000000000, 1.000000000000000000 ) ) ;
#5404=EDGE_CURVE ( 'NONE', #2540, #4041, #1159, .T. ) ;
#5412=EDGE_CURVE ( 'NONE', #8113, #4311, #6005, .T. ) ;
#5423=CIRCLE ( 'NONE', #6555, 2.149999999999985256 ) ;
#5424=ADVANCED_FACE ( 'NONE', ( #3855 ), #483, .F. ) ;
#5436=EDGE_LOOP ( 'NONE', ( #8272, #6119 ) ) ;
#5467=CARTESIAN_POINT ( 'NONE',  ( 39.85000000000002274, -21.99999999999992184, 60.00000000000002842 ) ) ;
#5469=DIRECTION ( 'NONE',  ( -0.000000000000000000, -0.000000000000000000, 1.000000000000000000 ) ) ;
#5491=EDGE_LOOP ( 'NONE', ( #3054, #6233 ) ) ;
#5523=ORIENTED_EDGE ( 'NONE', *, *, #4679, .F. ) ;
#5530=ORIENTED_EDGE ( 'NONE', *, *, #1421, .F. ) ;
#5578=VERTEX_POINT ( 'NONE', #1376 ) ;
#5585=FILL_AREA_STYLE ('',( #2120 ) ) ;
#5601=DIRECTION ( 'NONE',  ( -0.000000000000000000, 0.000000000000000000, 1.000000000000000000 ) ) ;
#5632=( NAMED_UNIT ( * ) PLANE_ANGLE_UNIT ( ) SI_UNIT ( $, .RADIAN. ) );
#5676=DIRECTION ( 'NONE',  ( -0.000000000000000000, -0.000000000000000000, 1.000000000000000000 ) ) ;
#5711=DIRECTION ( 'NONE',  ( -0.000000000000000000, -0.000000000000000000, 1.000000000000000000 ) ) ;
#5720=DIRECTION ( 'NONE',  ( -0.000000000000000000, 0.000000000000000000, 1.000000000000000000 ) ) ;
#5723=AXIS2_PLACEMENT_3D ( 'NONE', #1383, #2008, #5386 ) ;
#5731=ADVANCED_FACE ( 'NONE', ( #3979, #7458, #2618, #6043, #1416, #4112, #8653 ), #7414, .F. ) ;
#5736=DIRECTION ( 'NONE',  ( -0.000000000000000000, -0.000000000000000000, 1.000000000000000000 ) ) ;
#5805=EDGE_LOOP ( 'NONE', ( #3823, #6205, #2007, #1136 ) ) ;
#5810=CARTESIAN_POINT ( 'NONE',  ( 39.85000000000002274, -21.99999999999992184, 80.00000000000002842 ) ) ;
#5814=ORIENTED_EDGE ( 'NONE', *, *, #6127, .T. ) ;
#5815=CIRCLE ( 'NONE', #5375, 2.149999999999985256 ) ;
#5818=ADVANCED_FACE ( 'NONE', ( #7324 ), #3326, .F. ) ;
#5848=ORIENTED_EDGE ( 'NONE', *, *, #7251, .F. ) ;
#5871=CARTESIAN_POINT ( 'NONE',  ( -50.00000000000002842, 30.00000000000000000, 80.00000000000002842 ) ) ;
#5886=EDGE_CURVE ( 'NONE', #2517, #120, #184, .T. ) ;
#5890=VERTEX_POINT ( 'NONE', #3017 ) ;
#5914=DIRECTION ( 'NONE',  ( 1.000000000000000000, 0.000000000000000000, -0.000000000000000000 ) ) ;
#5921=CIRCLE ( 'NONE', #7471, 9.999999999999994671 ) ;
#5926=CARTESIAN_POINT ( 'NONE',  ( -50.00000000000002842, -30.00000000000000000, 80.00000000000002842 ) ) ;
#5940=ORIENTED_EDGE ( 'NONE', *, *, #3384, .T. ) ;
#5943=VECTOR ( 'NONE', #8018, 1000.000000000000000 ) ;
#5944=CYLINDRICAL_SURFACE ( 'NONE', #2952, 9.999999999999994671 ) ;
#5945=DIRECTION ( 'NONE',  ( -0.000000000000000000, -0.000000000000000000, 1.000000000000000000 ) ) ;
#5958=VERTEX_POINT ( 'NONE', #6179 ) ;
#5963=DIRECTION ( 'NONE',  ( -0.000000000000000000, 0.000000000000000000, 1.000000000000000000 ) ) ;
#5970=FACE_OUTER_BOUND ( 'NONE', #5805, .T. ) ;
#5981=DIRECTION ( 'NONE',  ( 1.000000000000000000, 0.000000000000000000, 0.000000000000000000 ) ) ;
#6000=DIRECTION ( 'NONE',  ( 1.000000000000000000, 0.000000000000000000, 0.000000000000000000 ) ) ;
#6005=CIRCLE ( 'NONE', #6707, 9.999999999999994671 ) ;
#6021=FACE_OUTER_BOUND ( 'NONE', #4385, .T. ) ;
#6025=LINE ( 'NONE', #4751, #1635 ) ;
#6030=ORIENTED_EDGE ( 'NONE', *, *, #7814, .T. ) ;
#6043=FACE_BOUND ( 'NONE', #7020, .T. ) ;
#6047=FACE_OUTER_BOUND ( 'NONE', #779, .T. ) ;
#6066=FACE_OUTER_BOUND ( 'NONE', #6433, .T. ) ;
#6094=FACE_OUTER_BOUND ( 'NONE', #4478, .T. ) ;
#6095=CARTESIAN_POINT ( 'NONE',  ( -20.00000000000000355, 0.000000000000000000, 80.00000000000002842 ) ) ;
#6098=CARTESIAN_POINT ( 'NONE',  ( 39.99999999999996447, 1.102182119232617753E-14, 80.00000000000002842 ) ) ;
#6119=ORIENTED_EDGE ( 'NONE', *, *, #5294, .T. ) ;
#6127=EDGE_CURVE ( 'NONE', #4984, #5890, #1778, .T. ) ;
#6131=ADVANCED_FACE ( 'NONE', ( #7058 ), #2480, .F. ) ;
#6135=ORIENTED_EDGE ( 'NONE', *, *, #4417, .T. ) ;
#6141=DIRECTION ( 'NONE',  ( -0.000000000000000000, -0.000000000000000000, 1.000000000000000000 ) ) ;
#6143=DIRECTION ( 'NONE',  ( 1.000000000000000000, 0.000000000000000000, 0.000000000000000000 ) ) ;
#6156=VERTEX_POINT ( 'NONE', #3838 ) ;
#6179=CARTESIAN_POINT ( 'NONE',  ( -44.14999999999995595, -22.00000000000000000, 60.00000000000002842 ) ) ;
#6205=ORIENTED_EDGE ( 'NONE', *, *, #4675, .F. ) ;
#6210=VECTOR ( 'NONE', #1230, 1000.000000000000000 ) ;
#6223=EDGE_CURVE ( 'NONE', #4124, #5183, #350, .T. ) ;
#6227=DIRECTION ( 'NONE',  ( -0.000000000000000000, -0.000000000000000000, 1.000000000000000000 ) ) ;
#6233=ORIENTED_EDGE ( 'NONE', *, *, #3138, .T. ) ;
#6234=CARTESIAN_POINT ( 'NONE',  ( 42.00000000000000711, 21.99999999999992184, 80.00000000000002842 ) ) ;
#6241=ORIENTED_EDGE ( 'NONE', *, *, #8591, .T. ) ;
#6262=ORIENTED_EDGE ( 'NONE', *, *, #2490, .F. ) ;
#6266=CARTESIAN_POINT ( 'NONE',  ( 42.00000000000000711, -21.99999999999992184, 60.00000000000002842 ) ) ;
#6281=EDGE_CURVE ( 'NONE', #923, #4984, #878, .T. ) ;
#6291=ORIENTED_EDGE ( 'NONE', *, *, #4407, .T. ) ;
#6312=LINE ( 'NONE', #3630, #3798 ) ;
#6314=DIRECTION ( 'NONE',  ( 1.000000000000000000, 0.000000000000000000, 0.000000000000000000 ) ) ;
#6333=ORIENTED_EDGE ( 'NONE', *, *, #4976, .T. ) ;
#6363=AXIS2_PLACEMENT_3D ( 'NONE', #874, #831, #4854 ) ;
#6370=CARTESIAN_POINT ( 'NONE',  ( 39.99999999999996447, 1.102182119232617753E-14, 60.00000000000002842 ) ) ;
#6381=DIRECTION ( 'NONE',  ( 1.000000000000000000, 0.000000000000000000, 0.000000000000000000 ) ) ;
#6382=EDGE_CURVE ( 'NONE', #2302, #8507, #3561, .T. ) ;
#6383=CARTESIAN_POINT ( 'NONE',  ( 29.99999999999997158, 1.102182119232617753E-14, 60.00000000000002842 ) ) ;
#6400=DIRECTION ( 'NONE',  ( 1.000000000000000000, 0.000000000000000000, 0.000000000000000000 ) ) ;
#6426=AXIS2_PLACEMENT_3D ( 'NONE', #3380, #1291, #3992 ) ;
#6432=AXIS2_PLACEMENT_3D ( 'NONE', #7739, #3116, #4472 ) ;
#6433=EDGE_LOOP ( 'NONE', ( #4612, #4519, #15, #1811 ) ) ;
#6472=ORIENTED_EDGE ( 'NONE', *, *, #250, .F. ) ;
#6474=AXIS2_PLACEMENT_3D ( 'NONE', #576, #670, #3291 ) ;
#6483=PLANE ( 'NONE',  #3147 ) ;
#6496=CARTESIAN_POINT ( 'NONE',  ( 42.00000000000000711, 21.99999999999992184, 80.00000000000002842 ) ) ;
#6534=DIRECTION ( 'NONE',  ( -0.000000000000000000, -0.000000000000000000, 1.000000000000000000 ) ) ;
#6544=VERTEX_POINT ( 'NONE', #7046 ) ;
#6545=ORIENTED_EDGE ( 'NONE', *, *, #7251, .T. ) ;
#6555=AXIS2_PLACEMENT_3D ( 'NONE', #8674, #2021, #3875 ) ;
#6556=AXIS2_PLACEMENT_3D ( 'NONE', #6234, #3596, #1104 ) ;
#6561=VECTOR ( 'NONE', #3895, 1000.000000000000000 ) ;
#6564=AXIS2_PLACEMENT_3D ( 'NONE', #5286, #7993, #662 ) ;
#6579=CARTESIAN_POINT ( 'NONE',  ( -20.00000000000000000, 0.000000000000000000, 80.00000000000002842 ) ) ;
#6581=( NAMED_UNIT ( * ) PLANE_ANGLE_UNIT ( ) SI_UNIT ( $, .RADIAN. ) );
#6589=DIRECTION ( 'NONE',  ( -0.000000000000000000, -0.000000000000000000, 1.000000000000000000 ) ) ;
#6619=LINE ( 'NONE', #2670, #8590 ) ;
#6641=DIRECTION ( 'NONE',  ( 1.000000000000000000, 0.000000000000000000, 0.000000000000000000 ) ) ;
#6659=APPLICATION_CONTEXT ( 'automotive_design' ) ;
#6663=DIRECTION ( 'NONE',  ( 1.000000000000000000, 0.000000000000000000, 0.000000000000000000 ) ) ;
#6676=EDGE_LOOP ( 'NONE', ( #6803, #6472, #6291, #770 ) ) ;
#6687=CIRCLE ( 'NONE', #1911, 9.999999999999998224 ) ;
#6706=CARTESIAN_POINT ( 'NONE',  ( 29.99999999999997158, 1.102182119232617753E-14, 80.00000000000002842 ) ) ;
#6707=AXIS2_PLACEMENT_3D ( 'NONE', #5049, #6534, #2413 ) ;
#6715=EDGE_LOOP ( 'NONE', ( #2819, #1886 ) ) ;
#6729=EDGE_CURVE ( 'NONE', #7212, #4697, #2304, .T. ) ;
#6742=DIRECTION ( 'NONE',  ( -0.000000000000000000, 0.000000000000000000, 1.000000000000000000 ) ) ;
#6779=AXIS2_PLACEMENT_3D ( 'NONE', #684, #2597, #4616 ) ;
#6798=FACE_OUTER_BOUND ( 'NONE', #8315, .T. ) ;
#6800=DIRECTION ( 'NONE',  ( 1.000000000000000000, 0.000000000000000000, 0.000000000000000000 ) ) ;
#6803=ORIENTED_EDGE ( 'NONE', *, *, #4940, .F. ) ;
#6821=SURFACE_STYLE_FILL_AREA ( #5585 ) ;
#6868=CARTESIAN_POINT ( 'NONE',  ( -41.99999999999996447, -22.00000000000000000, 80.00000000000002842 ) ) ;
#6872=ADVANCED_FACE ( 'NONE', ( #5227 ), #7258, .F. ) ;
#6894=VECTOR ( 'NONE', #5469, 1000.000000000000000 ) ;
#6899=CIRCLE ( 'NONE', #3536, 2.149999999999985256 ) ;
#6909=CARTESIAN_POINT ( 'NONE',  ( 50.00000000000002842, -30.00000000000000000, 60.00000000000002842 ) ) ;
#6914=ORIENTED_EDGE ( 'NONE', *, *, #6382, .F. ) ;
#6936=AXIS2_PLACEMENT_3D ( 'NONE', #67, #1929, #8670 ) ;
#6965=DIRECTION ( 'NONE',  ( -0.000000000000000000, 0.000000000000000000, 1.000000000000000000 ) ) ;
#7020=EDGE_LOOP ( 'NONE', ( #1350, #680 ) ) ;
#7021=FACE_OUTER_BOUND ( 'NONE', #8244, .T. ) ;
#7029=DIRECTION ( 'NONE',  ( -0.000000000000000000, -0.000000000000000000, 1.000000000000000000 ) ) ;
#7046=CARTESIAN_POINT ( 'NONE',  ( -39.84999999999998010, -22.00000000000000000, 60.00000000000002842 ) ) ;
#7052=CIRCLE ( 'NONE', #1712, 2.149999999999985256 ) ;
#7058=FACE_OUTER_BOUND ( 'NONE', #7745, .T. ) ;
#7060=DIRECTION ( 'NONE',  ( 1.000000000000000000, 0.000000000000000000, 0.000000000000000000 ) ) ;
#7071=ORIENTED_EDGE ( 'NONE', *, *, #6281, .T. ) ;
#7080=DIRECTION ( 'NONE',  ( -0.000000000000000000, -0.000000000000000000, 1.000000000000000000 ) ) ;
#7090=DIRECTION ( 'NONE',  ( 1.000000000000000000, 0.000000000000000000, 0.000000000000000000 ) ) ;
#7098=CIRCLE ( 'NONE', #3308, 2.149999999999985256 ) ;
#7151=ORIENTED_EDGE ( 'NONE', *, *, #2496, .T. ) ;
#7170=CARTESIAN_POINT ( 'NONE',  ( -41.99999999999996447, -22.00000000000000000, 60.00000000000002842 ) ) ;
#7185=CARTESIAN_POINT ( 'NONE',  ( -41.99999999999996447, 22.00000000000000000, 80.00000000000002842 ) ) ;
#7187=CARTESIAN_POINT ( 'NONE',  ( 50.00000000000002842, 30.00000000000000000, 80.00000000000002842 ) ) ;
#7190=( GEOMETRIC_REPRESENTATION_CONTEXT ( 3 ) GLOBAL_UNCERTAINTY_ASSIGNED_CONTEXT ( ( #608 ) ) GLOBAL_UNIT_ASSIGNED_CONTEXT ( ( #1837, #3246, #2628 ) ) REPRESENTATION_CONTEXT ( 'NONE', 'WORKASPACE' ) );
#7212=VERTEX_POINT ( 'NONE', #6370 ) ;
#7219=EDGE_LOOP ( 'NONE', ( #4977, #8220, #642, #3527 ) ) ;
#7233=DIRECTION ( 'NONE',  ( 1.000000000000000000, 0.000000000000000000, 0.000000000000000000 ) ) ;
#7240=LINE ( 'NONE', #4599, #6561 ) ;
#7251=EDGE_CURVE ( 'NONE', #1887, #5183, #7098, .T. ) ;
#7258=CYLINDRICAL_SURFACE ( 'NONE', #4121, 2.149999999999985256 ) ;
#7270=LINE ( 'NONE', #7891, #6210 ) ;
#7296=EDGE_LOOP ( 'NONE', ( #7920, #2913, #7516, #2071 ) ) ;
#7321=DIRECTION ( 'NONE',  ( 1.000000000000000000, 0.000000000000000000, 0.000000000000000000 ) ) ;
#7323=ORIENTED_EDGE ( 'NONE', *, *, #2930, .F. ) ;
#7324=FACE_OUTER_BOUND ( 'NONE', #6676, .T. ) ;
#7327=FACE_BOUND ( 'NONE', #48, .T. ) ;
#7350=EDGE_LOOP ( 'NONE', ( #4321, #6241 ) ) ;
#7379=DIRECTION ( 'NONE',  ( 0.000000000000000000, -1.000000000000000000, 0.000000000000000000 ) ) ;
#7382=VERTEX_POINT ( 'NONE', #6579 ) ;
#7394=FACE_OUTER_BOUND ( 'NONE', #3904, .T. ) ;
#7414=PLANE ( 'NONE',  #6564 ) ;
#7432=ORIENTED_EDGE ( 'NONE', *, *, #8448, .F. ) ;
#7434=CYLINDRICAL_SURFACE ( 'NONE', #6936, 2.149999999999985256 ) ;
#7457=VERTEX_POINT ( 'NONE', #5926 ) ;
#7458=FACE_BOUND ( 'NONE', #5436, .T. ) ;
#7471=AXIS2_PLACEMENT_3D ( 'NONE', #2437, #6965, #7722 ) ;
#7483=VERTEX_POINT ( 'NONE', #5177 ) ;
#7516=ORIENTED_EDGE ( 'NONE', *, *, #3878, .T. ) ;
#7527=EDGE_LOOP ( 'NONE', ( #3385, #108 ) ) ;
#7545=LINE ( 'NONE', #6095, #6894 ) ;
#7585=CARTESIAN_POINT ( 'NONE',  ( 50.00000000000002842, -30.00000000000000000, 80.00000000000002842 ) ) ;
#7586=EDGE_CURVE ( 'NONE', #4648, #1297, #3203, .T. ) ;
#7672=DIRECTION ( 'NONE',  ( 1.000000000000000000, 0.000000000000000000, 0.000000000000000000 ) ) ;
#7676=PRODUCT ( 'guide block', 'guide block', '', ( #4727 ) ) ;
#7694=EDGE_CURVE ( 'NONE', #7212, #8113, #3594, .T. ) ;
#7722=DIRECTION ( 'NONE',  ( 1.000000000000000000, 0.000000000000000000, 0.000000000000000000 ) ) ;
#7730=LINE ( 'NONE', #8440, #4332 ) ;
#7739=CARTESIAN_POINT ( 'NONE',  ( 50.00000000000002842, 30.00000000000000000, 80.00000000000002842 ) ) ;
#7741=CARTESIAN_POINT ( 'NONE',  ( -41.99999999999996447, 22.00000000000000000, 80.00000000000002842 ) ) ;
#7745=EDGE_LOOP ( 'NONE', ( #4265, #2447, #5814, #5940 ) ) ;
#7769=DIRECTION ( 'NONE',  ( -0.000000000000000000, -0.000000000000000000, 1.000000000000000000 ) ) ;
#7780=CARTESIAN_POINT ( 'NONE',  ( 44.14999999999999147, -21.99999999999992184, 80.00000000000002842 ) ) ;
#7787=CARTESIAN_POINT ( 'NONE',  ( 0.000000000000000000, 0.000000000000000000, 0.000000000000000000 ) ) ;
#7814=EDGE_CURVE ( 'NONE', #8507, #2302, #5815, .T. ) ;
#7819=ORIENTED_EDGE ( 'NONE', *, *, #1421, .T. ) ;
#7848=STYLED_ITEM ( 'NONE', ( #2957 ), #85 ) ;
#7853=APPLICATION_CONTEXT ( 'automotive_design' ) ;
#7856=DIRECTION ( 'NONE',  ( -0.000000000000000000, -0.000000000000000000, 1.000000000000000000 ) ) ;
#7858=ADVANCED_FACE ( 'NONE', ( #4633 ), #6483, .F. ) ;
#7864=VECTOR ( 'NONE', #2252, 1000.000000000000000 ) ;
#7877=EDGE_LOOP ( 'NONE', ( #2604, #1894, #6030, #851 ) ) ;
#7891=CARTESIAN_POINT ( 'NONE',  ( -50.00000000000002842, 30.00000000000000000, 60.00000000000002842 ) ) ;
#7912=CARTESIAN_POINT ( 'NONE',  ( -50.00000000000002842, 30.00000000000000000, 60.00000000000002842 ) ) ;
#7920=ORIENTED_EDGE ( 'NONE', *, *, #4106, .F. ) ;
#7929=EDGE_LOOP ( 'NONE', ( #8470, #2187 ) ) ;
#7956=SURFACE_STYLE_USAGE ( .BOTH. , #3295 ) ;
#7975=VECTOR ( 'NONE', #5000, 1000.000000000000000 ) ;
#7992=ORIENTED_EDGE ( 'NONE', *, *, #2313, .F. ) ;
#7993=DIRECTION ( 'NONE',  ( -0.000000000000000000, 0.000000000000000000, 1.000000000000000000 ) ) ;
#7997=DIRECTION ( 'NONE',  ( -0.000000000000000000, -0.000000000000000000, 1.000000000000000000 ) ) ;
#8000=CARTESIAN_POINT ( 'NONE',  ( 42.00000000000000711, -21.99999999999992184, 80.00000000000002842 ) ) ;
#8012=CYLINDRICAL_SURFACE ( 'NONE', #6779, 9.999999999999994671 ) ;
#8018=DIRECTION ( 'NONE',  ( -0.000000000000000000, -0.000000000000000000, 1.000000000000000000 ) ) ;
#8028=UNCERTAINTY_MEASURE_WITH_UNIT (LENGTH_MEASURE( 1.000000000000000082E-05 ), #490, 'distance_accuracy_value', 'NONE');
#8056=CARTESIAN_POINT ( 'NONE',  ( -41.99999999999996447, -22.00000000000000000, 80.00000000000002842 ) ) ;
#8057=DIRECTION ( 'NONE',  ( 0.000000000000000000, 1.000000000000000000, 0.000000000000000000 ) ) ;
#8104=EDGE_CURVE ( 'NONE', #6156, #2506, #5921, .T. ) ;
#8113=VERTEX_POINT ( 'NONE', #4239 ) ;
#8169=AXIS2_PLACEMENT_3D ( 'NONE', #1780, #7769, #6400 ) ;
#8172=EDGE_LOOP ( 'NONE', ( #994, #7071 ) ) ;
#8176=VECTOR ( 'NONE', #938, 1000.000000000000000 ) ;
#8192=ORIENTED_EDGE ( 'NONE', *, *, #1854, .T. ) ;
#8199=EDGE_CURVE ( 'NONE', #2072, #2540, #7052, .T. ) ;
#8220=ORIENTED_EDGE ( 'NONE', *, *, #1854, .F. ) ;
#8244=EDGE_LOOP ( 'NONE', ( #5356, #2189, #436, #6545 ) ) ;
#8264=CARTESIAN_POINT ( 'NONE',  ( 19.99999999999997513, 1.224646799147352901E-14, 80.00000000000002842 ) ) ;
#8272=ORIENTED_EDGE ( 'NONE', *, *, #6729, .T. ) ;
#8315=EDGE_LOOP ( 'NONE', ( #5025, #8455, #4253, #4919 ) ) ;
#8331=( NAMED_UNIT ( * ) SI_UNIT ( $, .STERADIAN. ) SOLID_ANGLE_UNIT ( ) );
#8394=PRODUCT_DEFINITION_SHAPE ( 'NONE', 'NONE',  #1576 ) ;
#8416=ORIENTED_EDGE ( 'NONE', *, *, #2490, .T. ) ;
#8419=AXIS2_PLACEMENT_3D ( 'NONE', #49, #2753, #6000 ) ;
#8440=CARTESIAN_POINT ( 'NONE',  ( -44.14999999999995595, -22.00000000000000000, 80.00000000000002842 ) ) ;
#8448=EDGE_CURVE ( 'NONE', #1297, #1434, #7270, .T. ) ;
#8455=ORIENTED_EDGE ( 'NONE', *, *, #6223, .T. ) ;
#8470=ORIENTED_EDGE ( 'NONE', *, *, #3384, .F. ) ;
#8474=COLOUR_RGB ( '', 0.09019608, 0.27058824, 0.51372549) ;
#8484=AXIS2_PLACEMENT_3D ( 'NONE', #6868, #4318, #80 ) ;
#8507=VERTEX_POINT ( 'NONE', #3835 ) ;
#8542=CARTESIAN_POINT ( 'NONE',  ( -44.14999999999995595, 22.00000000000000000, 80.00000000000002842 ) ) ;
#8552=PRODUCT_DEFINITION_CONTEXT ( 'detailed design', #6659, 'design' ) ;
#8582=CARTESIAN_POINT ( 'NONE',  ( 50.00000000000002842, -30.00000000000000000, 80.00000000000002842 ) ) ;
#8590=VECTOR ( 'NONE', #4604, 1000.000000000000000 ) ;
#8591=EDGE_CURVE ( 'NONE', #4124, #3192, #4941, .T. ) ;
#8617=DIRECTION ( 'NONE',  ( 1.000000000000000000, 0.000000000000000000, 0.000000000000000000 ) ) ;
#8638=ORIENTED_EDGE ( 'NONE', *, *, #5294, .F. ) ;
#8639=LINE ( 'NONE', #1685, #1060 ) ;
#8653=FACE_OUTER_BOUND ( 'NONE', #234, .T. ) ;
#8667=ORIENTED_EDGE ( 'NONE', *, *, #2313, .T. ) ;
#8670=DIRECTION ( 'NONE',  ( 1.000000000000000000, 0.000000000000000000, 0.000000000000000000 ) ) ;
#8674=CARTESIAN_POINT ( 'NONE',  ( 42.00000000000000711, -21.99999999999992184, 60.00000000000002842 ) ) ;
#8684=AXIS2_PLACEMENT_3D ( 'NONE', #7170, #1131, #2386 ) ;
#8694=FACE_OUTER_BOUND ( 'NONE', #2680, .T. ) ;
ENDSEC;
END-ISO-10303-21;
